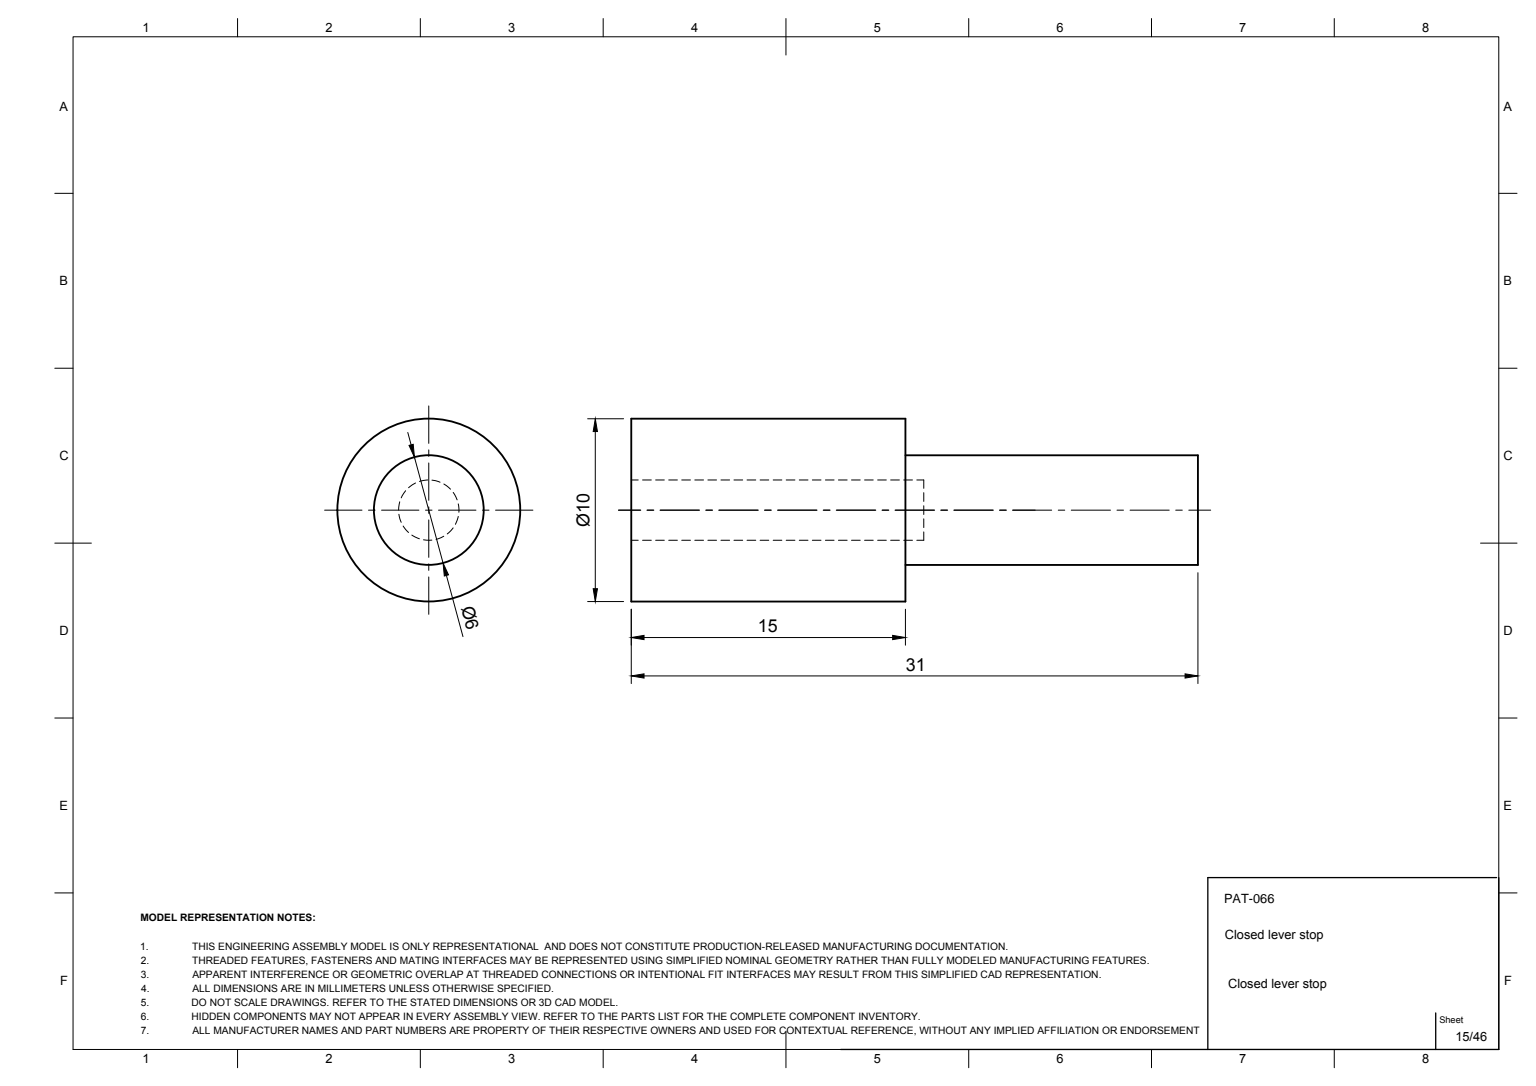
ISO-10303-21;
HEADER;
/* Generated by software containing ST-Developer
 * from STEP Tools, Inc. (www.steptools.com) 
 */

FILE_DESCRIPTION(
/* description */ ('Lever-operated bar clamp (toggle)'),
/* implementation_level */ '2;1');

FILE_NAME(
/* name */ 'Closed lever stop.step',
/* time_stamp */ '2026-10-28T03:25:02-07:00',
/* author */ (''),
/* organization */ (''),
/* preprocessor_version */ 'ST-DEVELOPER v20.2',
/* originating_system */ 'Autodesk Translation Framework v15.17.0.0',
/* authorisation */ '');

FILE_SCHEMA (('AUTOMOTIVE_DESIGN { 1 0 10303 214 3 1 1 }'));
ENDSEC;

DATA;
#10=MECHANICAL_DESIGN_GEOMETRIC_PRESENTATION_REPRESENTATION('',(#420),#12413);
#344=SHAPE_REPRESENTATION_RELATIONSHIP('SRR','None',#12583,#382);
#382=ADVANCED_BREP_SHAPE_REPRESENTATION('',(#467),#12380);
#420=STYLED_ITEM('',(#12862),#467);
#467=MANIFOLD_SOLID_BREP('Body1',#6579);
#585=FACE_BOUND('',#1510,.T.);
#586=FACE_BOUND('',#1513,.T.);
#724=PLANE('',#7293);
#725=PLANE('',#7294);
#726=PLANE('',#7299);
#727=PLANE('',#7302);
#1016=FACE_OUTER_BOUND('',#1507,.T.);
#1017=FACE_OUTER_BOUND('',#1508,.T.);
#1018=FACE_OUTER_BOUND('',#1509,.T.);
#1019=FACE_OUTER_BOUND('',#1511,.T.);
#1020=FACE_OUTER_BOUND('',#1512,.T.);
#1021=FACE_OUTER_BOUND('',#1514,.T.);
#1022=FACE_OUTER_BOUND('',#1515,.T.);
#1507=EDGE_LOOP('',(#4967,#4968,#4969,#4970));
#1508=EDGE_LOOP('',(#4971));
#1509=EDGE_LOOP('',(#4972));
#1510=EDGE_LOOP('',(#4973));
#1511=EDGE_LOOP('',(#4974,#4975,#4976,#4977));
#1512=EDGE_LOOP('',(#4978));
#1513=EDGE_LOOP('',(#4979));
#1514=EDGE_LOOP('',(#4980,#4981,#4982,#4983));
#1515=EDGE_LOOP('',(#4984));
#2014=LINE('',#10645,#2455);
#2015=LINE('',#10656,#2456);
#2016=LINE('',#10660,#2457);
#2455=VECTOR('',#8563,0.165);
#2456=VECTOR('',#8578,0.5);
#2457=VECTOR('',#8583,0.3);
#2843=CIRCLE('',#7291,0.165);
#2844=CIRCLE('',#7292,0.165);
#2845=CIRCLE('',#7295,0.5);
#2846=CIRCLE('',#7296,0.3);
#2847=CIRCLE('',#7298,0.5);
#2848=CIRCLE('',#7301,0.3);
#3256=VERTEX_POINT('',#10642);
#3257=VERTEX_POINT('',#10644);
#3258=VERTEX_POINT('',#10649);
#3259=VERTEX_POINT('',#10651);
#3260=VERTEX_POINT('',#10654);
#3261=VERTEX_POINT('',#10659);
#3888=EDGE_CURVE('',#3256,#3256,#2843,.T.);
#3889=EDGE_CURVE('',#3256,#3257,#2014,.T.);
#3890=EDGE_CURVE('',#3257,#3257,#2844,.T.);
#3891=EDGE_CURVE('',#3258,#3258,#2845,.T.);
#3892=EDGE_CURVE('',#3259,#3259,#2846,.T.);
#3893=EDGE_CURVE('',#3260,#3260,#2847,.T.);
#3894=EDGE_CURVE('',#3260,#3258,#2015,.T.);
#3895=EDGE_CURVE('',#3259,#3261,#2016,.T.);
#3896=EDGE_CURVE('',#3261,#3261,#2848,.T.);
#4967=ORIENTED_EDGE('',*,*,#3888,.F.);
#4968=ORIENTED_EDGE('',*,*,#3889,.T.);
#4969=ORIENTED_EDGE('',*,*,#3890,.F.);
#4970=ORIENTED_EDGE('',*,*,#3889,.F.);
#4971=ORIENTED_EDGE('',*,*,#3888,.T.);
#4972=ORIENTED_EDGE('',*,*,#3891,.F.);
#4973=ORIENTED_EDGE('',*,*,#3892,.T.);
#4974=ORIENTED_EDGE('',*,*,#3893,.F.);
#4975=ORIENTED_EDGE('',*,*,#3894,.T.);
#4976=ORIENTED_EDGE('',*,*,#3891,.T.);
#4977=ORIENTED_EDGE('',*,*,#3894,.F.);
#4978=ORIENTED_EDGE('',*,*,#3893,.T.);
#4979=ORIENTED_EDGE('',*,*,#3890,.T.);
#4980=ORIENTED_EDGE('',*,*,#3892,.F.);
#4981=ORIENTED_EDGE('',*,*,#3895,.T.);
#4982=ORIENTED_EDGE('',*,*,#3896,.T.);
#4983=ORIENTED_EDGE('',*,*,#3895,.F.);
#4984=ORIENTED_EDGE('',*,*,#3896,.F.);
#6088=CYLINDRICAL_SURFACE('',#7290,0.165);
#6089=CYLINDRICAL_SURFACE('',#7297,0.5);
#6090=CYLINDRICAL_SURFACE('',#7300,0.3);
#6291=ADVANCED_FACE('',(#1016),#6088,.F.);
#6292=ADVANCED_FACE('',(#1017),#724,.T.);
#6293=ADVANCED_FACE('',(#1018,#585),#725,.F.);
#6294=ADVANCED_FACE('',(#1019),#6089,.T.);
#6295=ADVANCED_FACE('',(#1020,#586),#726,.T.);
#6296=ADVANCED_FACE('',(#1021),#6090,.T.);
#6297=ADVANCED_FACE('',(#1022),#727,.F.);
#6579=CLOSED_SHELL('',(#6291,#6292,#6293,#6294,#6295,#6296,#6297));
#7289=AXIS2_PLACEMENT_3D('',#10640,#8557,#8558);
#7290=AXIS2_PLACEMENT_3D('',#10641,#8559,#8560);
#7291=AXIS2_PLACEMENT_3D('',#10643,#8561,#8562);
#7292=AXIS2_PLACEMENT_3D('',#10646,#8564,#8565);
#7293=AXIS2_PLACEMENT_3D('',#10647,#8566,#8567);
#7294=AXIS2_PLACEMENT_3D('',#10648,#8568,#8569);
#7295=AXIS2_PLACEMENT_3D('',#10650,#8570,#8571);
#7296=AXIS2_PLACEMENT_3D('',#10652,#8572,#8573);
#7297=AXIS2_PLACEMENT_3D('',#10653,#8574,#8575);
#7298=AXIS2_PLACEMENT_3D('',#10655,#8576,#8577);
#7299=AXIS2_PLACEMENT_3D('',#10657,#8579,#8580);
#7300=AXIS2_PLACEMENT_3D('',#10658,#8581,#8582);
#7301=AXIS2_PLACEMENT_3D('',#10661,#8584,#8585);
#7302=AXIS2_PLACEMENT_3D('',#10662,#8586,#8587);
#8557=DIRECTION('axis',(0.,0.,1.));
#8558=DIRECTION('refdir',(1.,0.,0.));
#8559=DIRECTION('center_axis',(0.,1.,0.));
#8560=DIRECTION('ref_axis',(1.,0.,0.));
#8561=DIRECTION('center_axis',(0.,1.,0.));
#8562=DIRECTION('ref_axis',(1.,0.,0.));
#8563=DIRECTION('',(0.,1.,0.));
#8564=DIRECTION('center_axis',(0.,-1.,0.));
#8565=DIRECTION('ref_axis',(1.,0.,0.));
#8566=DIRECTION('center_axis',(0.,1.,0.));
#8567=DIRECTION('ref_axis',(1.,0.,0.));
#8568=DIRECTION('center_axis',(0.,1.,0.));
#8569=DIRECTION('ref_axis',(1.,0.,0.));
#8570=DIRECTION('center_axis',(0.,1.,0.));
#8571=DIRECTION('ref_axis',(1.,0.,0.));
#8572=DIRECTION('center_axis',(0.,1.,0.));
#8573=DIRECTION('ref_axis',(1.,0.,0.));
#8574=DIRECTION('center_axis',(0.,1.,0.));
#8575=DIRECTION('ref_axis',(1.,0.,0.));
#8576=DIRECTION('center_axis',(0.,1.,0.));
#8577=DIRECTION('ref_axis',(1.,0.,0.));
#8578=DIRECTION('',(0.,-1.,0.));
#8579=DIRECTION('center_axis',(0.,1.,0.));
#8580=DIRECTION('ref_axis',(1.,0.,0.));
#8581=DIRECTION('center_axis',(0.,1.,0.));
#8582=DIRECTION('ref_axis',(1.,0.,0.));
#8583=DIRECTION('',(0.,-1.,0.));
#8584=DIRECTION('center_axis',(0.,1.,0.));
#8585=DIRECTION('ref_axis',(1.,0.,0.));
#8586=DIRECTION('center_axis',(0.,1.,0.));
#8587=DIRECTION('ref_axis',(1.,0.,0.));
#10640=CARTESIAN_POINT('',(0.,0.,0.));
#10641=CARTESIAN_POINT('Origin',(-5.25982293614231,-2.4,14.8604204653858));
#10642=CARTESIAN_POINT('',(-5.42482293614231,-2.4,14.8604204653858));
#10643=CARTESIAN_POINT('Origin',(-5.25982293614231,-2.4,14.8604204653858));
#10644=CARTESIAN_POINT('',(-5.42482293614231,-0.8,14.8604204653858));
#10645=CARTESIAN_POINT('',(-5.42482293614231,-2.4,14.8604204653858));
#10646=CARTESIAN_POINT('Origin',(-5.25982293614231,-0.8,14.8604204653858));
#10647=CARTESIAN_POINT('Origin',(-5.25982293614231,-2.4,14.8604204653858));
#10648=CARTESIAN_POINT('Origin',(-5.25982293614231,-2.3,14.8604204653858));
#10649=CARTESIAN_POINT('',(-5.75982293614231,-2.3,14.8604204653858));
#10650=CARTESIAN_POINT('Origin',(-5.25982293614231,-2.3,14.8604204653858));
#10651=CARTESIAN_POINT('',(-5.55982293614231,-2.3,14.8604204653858));
#10652=CARTESIAN_POINT('Origin',(-5.25982293614231,-2.3,14.8604204653858));
#10653=CARTESIAN_POINT('Origin',(-5.25982293614231,-2.3,14.8604204653858));
#10654=CARTESIAN_POINT('',(-5.75982293614231,-0.8,14.8604204653858));
#10655=CARTESIAN_POINT('Origin',(-5.25982293614231,-0.8,14.8604204653858));
#10656=CARTESIAN_POINT('',(-5.75982293614231,-2.3,14.8604204653858));
#10657=CARTESIAN_POINT('Origin',(-5.25982293614231,-0.8,14.8604204653858));
#10658=CARTESIAN_POINT('Origin',(-5.25982293614231,-3.9,14.8604204653858));
#10659=CARTESIAN_POINT('',(-5.55982293614231,-3.9,14.8604204653858));
#10660=CARTESIAN_POINT('',(-5.55982293614231,-3.9,14.8604204653858));
#10661=CARTESIAN_POINT('Origin',(-5.25982293614231,-3.9,14.8604204653858));
#10662=CARTESIAN_POINT('Origin',(-5.25982293614231,-3.9,14.8604204653858));
#12334=UNCERTAINTY_MEASURE_WITH_UNIT(LENGTH_MEASURE(0.001),#12414,
'DISTANCE_ACCURACY_VALUE',
'Maximum model space distance between geometric entities at asserted c
onnectivities');
#12367=UNCERTAINTY_MEASURE_WITH_UNIT(LENGTH_MEASURE(0.001),#12414,
'DISTANCE_ACCURACY_VALUE',
'Maximum model space distance between geometric entities at asserted c
onnectivities');
#12380=(
GEOMETRIC_REPRESENTATION_CONTEXT(3)
GLOBAL_UNCERTAINTY_ASSIGNED_CONTEXT((#12334))
GLOBAL_UNIT_ASSIGNED_CONTEXT((#12414,#12416,#12417))
REPRESENTATION_CONTEXT('','3D')
);
#12413=(
GEOMETRIC_REPRESENTATION_CONTEXT(3)
GLOBAL_UNCERTAINTY_ASSIGNED_CONTEXT((#12367))
GLOBAL_UNIT_ASSIGNED_CONTEXT((#12414,#12416,#12417))
REPRESENTATION_CONTEXT('','3D')
);
#12414=(
LENGTH_UNIT()
NAMED_UNIT(*)
SI_UNIT(.CENTI.,.METRE.)
);
#12416=(
NAMED_UNIT(*)
PLANE_ANGLE_UNIT()
SI_UNIT($,.RADIAN.)
);
#12417=(
NAMED_UNIT(*)
SI_UNIT($,.STERADIAN.)
SOLID_ANGLE_UNIT()
);
#12430=SHAPE_DEFINITION_REPRESENTATION(#12475,#12583);
#12475=PRODUCT_DEFINITION_SHAPE('',$,#12629);
#12583=SHAPE_REPRESENTATION('',(#7289),#12380);
#12616=PRODUCT_DEFINITION_CONTEXT('part definition',#12753,'design');
#12629=PRODUCT_DEFINITION('Closed lever stop','Closed lever stop',#12674,
#12616);
#12674=PRODUCT_DEFINITION_FORMATION('',$,#12767);
#12753=APPLICATION_CONTEXT(
'Core Data for Automotive Mechanical Design Process');
#12754=PRODUCT_CONTEXT('part definition',#12753,'mechanical');
#12767=PRODUCT('Closed lever stop','Closed lever stop',
'Closed lever stop',(#12754));
#12856=COLOUR_RGB('Sky Blue',0.24,0.69,0.87);
#12857=FILL_AREA_STYLE_COLOUR('',#12856);
#12858=FILL_AREA_STYLE('',(#12857));
#12859=SURFACE_STYLE_FILL_AREA(#12858);
#12860=SURFACE_SIDE_STYLE('',(#12859));
#12861=SURFACE_STYLE_USAGE(.BOTH.,#12860);
#12862=PRESENTATION_STYLE_ASSIGNMENT((#12861));
ENDSEC;
END-ISO-10303-21;
